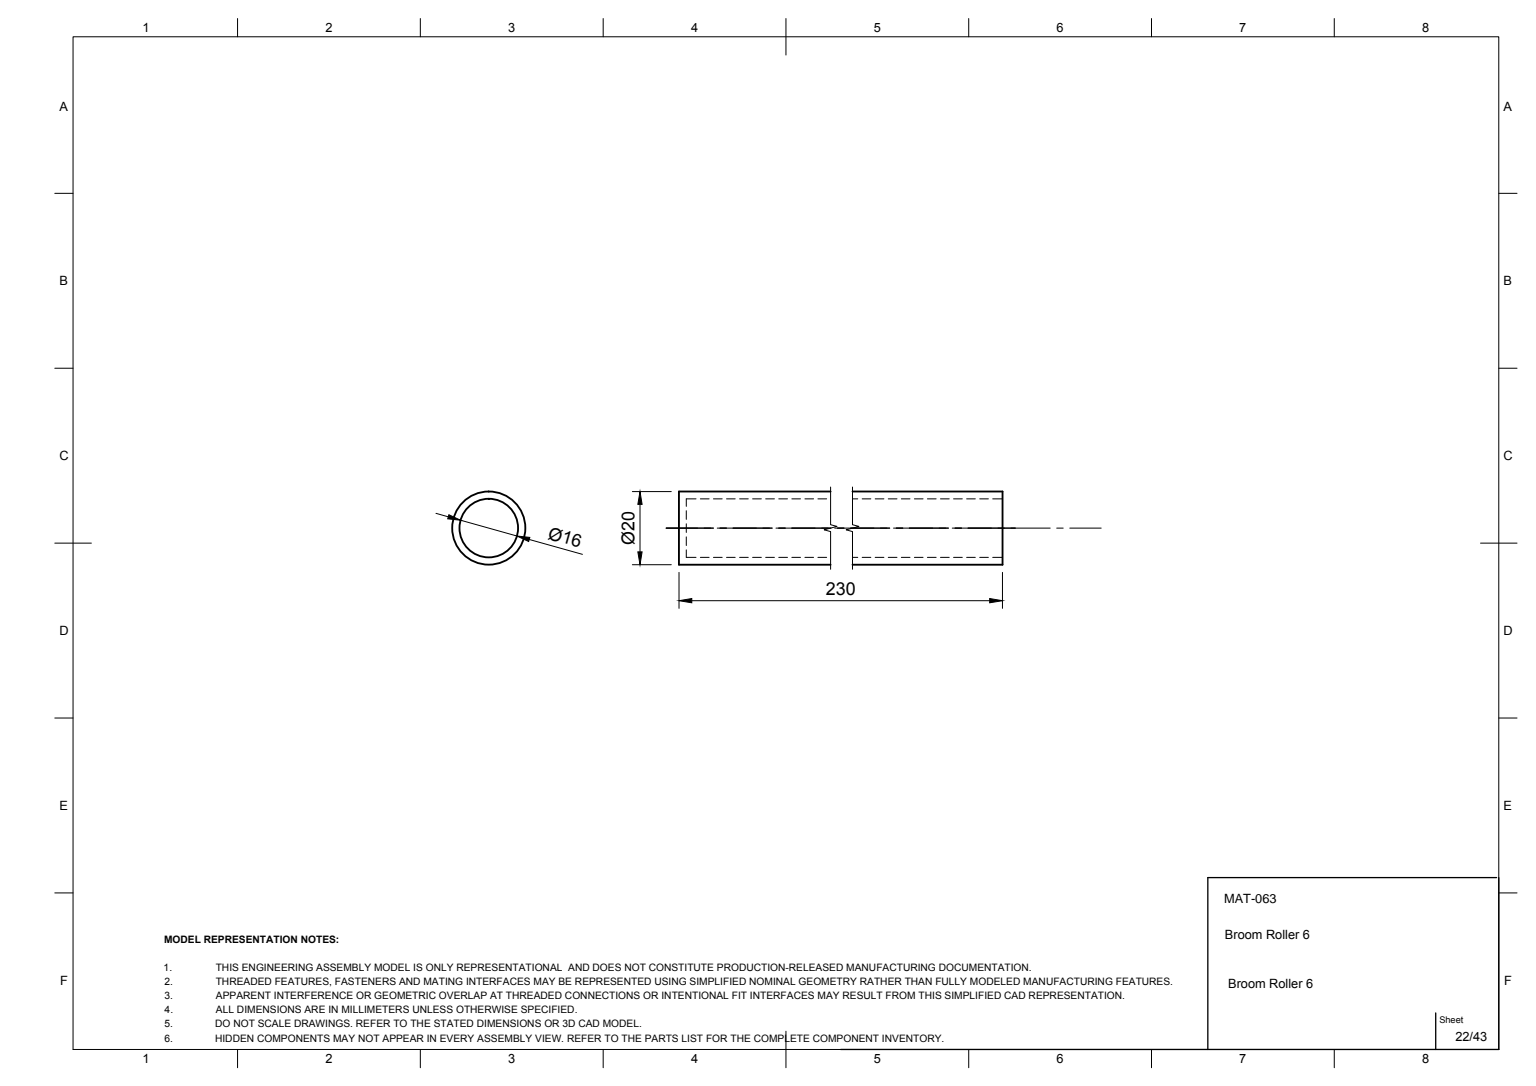
ISO-10303-21;
HEADER;
/* Generated by software containing ST-Developer
 * from STEP Tools, Inc. (www.steptools.com) 
 */

FILE_DESCRIPTION(
/* description */ (''),
/* implementation_level */ '2;1');

FILE_NAME(
/* name */ 'Broom Roller 6.step',
/* time_stamp */ '2026-10-24T09:43:01-07:00',
/* author */ (''),
/* organization */ (''),
/* preprocessor_version */ 'ST-DEVELOPER v20.2',
/* originating_system */ 'Autodesk Translation Framework v15.15.0.0',
/* authorisation */ '');

FILE_SCHEMA (('AUTOMOTIVE_DESIGN { 1 0 10303 214 3 1 1 }'));
ENDSEC;

DATA;
#10=MECHANICAL_DESIGN_GEOMETRIC_PRESENTATION_REPRESENTATION('',(#287),#11112);
#221=SHAPE_REPRESENTATION_RELATIONSHIP('SRR','None',#11245,#254);
#254=ADVANCED_BREP_SHAPE_REPRESENTATION('',(#320),#11090);
#287=STYLED_ITEM('',(#11426),#320);
#320=MANIFOLD_SOLID_BREP('Broom Roller 6',#6024);
#414=FACE_BOUND('',#1328,.T.);
#585=PLANE('',#6918);
#586=PLANE('',#6919);
#587=PLANE('',#6923);
#886=FACE_OUTER_BOUND('',#1325,.T.);
#887=FACE_OUTER_BOUND('',#1326,.T.);
#888=FACE_OUTER_BOUND('',#1327,.T.);
#889=FACE_OUTER_BOUND('',#1329,.T.);
#890=FACE_OUTER_BOUND('',#1330,.T.);
#1325=EDGE_LOOP('',(#4853,#4854,#4855,#4856));
#1326=EDGE_LOOP('',(#4857));
#1327=EDGE_LOOP('',(#4858));
#1328=EDGE_LOOP('',(#4859));
#1329=EDGE_LOOP('',(#4860,#4861,#4862,#4863));
#1330=EDGE_LOOP('',(#4864));
#1730=LINE('',#10291,#2089);
#1731=LINE('',#10300,#2090);
#2089=VECTOR('',#8452,0.00799999974106502);
#2090=VECTOR('',#8465,0.00999999987547767);
#2554=CIRCLE('',#6916,0.00799999974106502);
#2555=CIRCLE('',#6917,0.00799999974106502);
#2556=CIRCLE('',#6920,0.00999999987547767);
#2557=CIRCLE('',#6922,0.00999999987547767);
#2964=VERTEX_POINT('',#10288);
#2965=VERTEX_POINT('',#10290);
#2966=VERTEX_POINT('',#10295);
#2967=VERTEX_POINT('',#10298);
#3630=EDGE_CURVE('',#2964,#2964,#2554,.T.);
#3631=EDGE_CURVE('',#2964,#2965,#1730,.T.);
#3632=EDGE_CURVE('',#2965,#2965,#2555,.F.);
#3633=EDGE_CURVE('',#2966,#2966,#2556,.T.);
#3634=EDGE_CURVE('',#2967,#2967,#2557,.F.);
#3635=EDGE_CURVE('',#2967,#2966,#1731,.T.);
#4853=ORIENTED_EDGE('',*,*,#3630,.F.);
#4854=ORIENTED_EDGE('',*,*,#3631,.T.);
#4855=ORIENTED_EDGE('',*,*,#3632,.F.);
#4856=ORIENTED_EDGE('',*,*,#3631,.F.);
#4857=ORIENTED_EDGE('',*,*,#3632,.T.);
#4858=ORIENTED_EDGE('',*,*,#3633,.F.);
#4859=ORIENTED_EDGE('',*,*,#3630,.T.);
#4860=ORIENTED_EDGE('',*,*,#3634,.T.);
#4861=ORIENTED_EDGE('',*,*,#3635,.T.);
#4862=ORIENTED_EDGE('',*,*,#3633,.T.);
#4863=ORIENTED_EDGE('',*,*,#3635,.F.);
#4864=ORIENTED_EDGE('',*,*,#3634,.F.);
#5575=CYLINDRICAL_SURFACE('',#6915,0.00799999974106502);
#5576=CYLINDRICAL_SURFACE('',#6921,0.00999999987547767);
#5859=ADVANCED_FACE('',(#886),#5575,.F.);
#5860=ADVANCED_FACE('',(#887),#585,.F.);
#5861=ADVANCED_FACE('',(#888,#414),#586,.F.);
#5862=ADVANCED_FACE('',(#889),#5576,.T.);
#5863=ADVANCED_FACE('',(#890),#587,.T.);
#6024=CLOSED_SHELL('',(#5859,#5860,#5861,#5862,#5863));
#6914=AXIS2_PLACEMENT_3D('',#10286,#8446,#8447);
#6915=AXIS2_PLACEMENT_3D('',#10287,#8448,#8449);
#6916=AXIS2_PLACEMENT_3D('',#10289,#8450,#8451);
#6917=AXIS2_PLACEMENT_3D('',#10292,#8453,#8454);
#6918=AXIS2_PLACEMENT_3D('',#10293,#8455,#8456);
#6919=AXIS2_PLACEMENT_3D('',#10294,#8457,#8458);
#6920=AXIS2_PLACEMENT_3D('',#10296,#8459,#8460);
#6921=AXIS2_PLACEMENT_3D('',#10297,#8461,#8462);
#6922=AXIS2_PLACEMENT_3D('',#10299,#8463,#8464);
#6923=AXIS2_PLACEMENT_3D('',#10301,#8466,#8467);
#8446=DIRECTION('axis',(0.,0.,1.));
#8447=DIRECTION('refdir',(1.,0.,0.));
#8448=DIRECTION('center_axis',(0.,-0.604097518460404,-0.796910401607346));
#8449=DIRECTION('ref_axis',(0.,0.796910401607346,-0.604097518460404));
#8450=DIRECTION('center_axis',(0.,-0.604097518460404,-0.796910401607346));
#8451=DIRECTION('ref_axis',(0.,0.796910401607346,-0.604097518460404));
#8452=DIRECTION('',(0.,-0.604097518460404,-0.796910401607346));
#8453=DIRECTION('center_axis',(0.,-0.604097518460404,-0.796910401607346));
#8454=DIRECTION('ref_axis',(0.,0.796910401607346,-0.604097518460404));
#8455=DIRECTION('center_axis',(-1.20725909381357E-16,-0.6040974946122,-0.796910419685465));
#8456=DIRECTION('ref_axis',(7.15152886696226E-32,0.796910419685465,-0.6040974946122));
#8457=DIRECTION('center_axis',(6.24224782272207E-17,-0.604097506757326,
-0.796910410478859));
#8458=DIRECTION('ref_axis',(-1.64388262168888E-33,0.796910410478859,-0.604097506757326));
#8459=DIRECTION('center_axis',(0.,-0.604097518460408,-0.796910401607343));
#8460=DIRECTION('ref_axis',(0.,0.796910401607343,-0.604097518460408));
#8461=DIRECTION('center_axis',(0.,-0.604097518460408,-0.796910401607343));
#8462=DIRECTION('ref_axis',(0.,0.796910401607343,-0.604097518460408));
#8463=DIRECTION('center_axis',(0.,-0.604097518460408,-0.796910401607343));
#8464=DIRECTION('ref_axis',(0.,0.796910401607343,-0.604097518460408));
#8465=DIRECTION('',(0.,0.604097518460408,0.796910401607343));
#8466=DIRECTION('center_axis',(-2.35801524345747E-16,-0.604097538134134,
-0.796910386693685));
#8467=DIRECTION('ref_axis',(2.53292576583338E-33,0.796910386693685,-0.604097538134134));
#10286=CARTESIAN_POINT('',(0.,0.,0.));
#10287=CARTESIAN_POINT('Origin',(0.,0.488942429,1.283289392));
#10288=CARTESIAN_POINT('',(-9.79717407607493E-19,0.482567145986908,1.28812217198258));
#10289=CARTESIAN_POINT('Origin',(0.,0.488942428993417,1.28328939199132));
#10290=CARTESIAN_POINT('',(-9.79717407607493E-19,0.344832912126902,1.10642660087645));
#10291=CARTESIAN_POINT('',(-9.79717407607493E-19,0.482567145993489,1.28812217199126));
#10292=CARTESIAN_POINT('Origin',(0.,0.351208195133414,1.10159382088519));
#10293=CARTESIAN_POINT('Origin',(-1.99493199737333E-19,0.351208195,1.1015938205));
#10294=CARTESIAN_POINT('Origin',(-1.56125112837913E-19,0.488942429,1.2832893925));
#10295=CARTESIAN_POINT('',(-1.22464678389777E-18,0.480973325166166,1.28933036721888));
#10296=CARTESIAN_POINT('Origin',(0.,0.488942429083005,1.2832893921095));
#10297=CARTESIAN_POINT('Origin',(0.,0.488942429,1.283289392));
#10298=CARTESIAN_POINT('',(-1.22464678389777E-18,0.342030896187977,1.10604097520234));
#10299=CARTESIAN_POINT('Origin',(0.,0.350000000104818,1.10000000009296));
#10300=CARTESIAN_POINT('',(-1.22464678389777E-18,0.48097332508316,1.28933036710938));
#10301=CARTESIAN_POINT('Origin',(-1.56125112837913E-19,0.35,1.1));
#11051=UNCERTAINTY_MEASURE_WITH_UNIT(LENGTH_MEASURE(1.E-5),#11113,
'DISTANCE_ACCURACY_VALUE',
'Maximum model space distance between geometric entities at asserted c
onnectivities');
#11073=UNCERTAINTY_MEASURE_WITH_UNIT(LENGTH_MEASURE(1.E-5),#11113,
'DISTANCE_ACCURACY_VALUE',
'Maximum model space distance between geometric entities at asserted c
onnectivities');
#11090=(
GEOMETRIC_REPRESENTATION_CONTEXT(3)
GLOBAL_UNCERTAINTY_ASSIGNED_CONTEXT((#11051))
GLOBAL_UNIT_ASSIGNED_CONTEXT((#11113,#11114,#11115))
REPRESENTATION_CONTEXT('','3D')
);
#11112=(
GEOMETRIC_REPRESENTATION_CONTEXT(3)
GLOBAL_UNCERTAINTY_ASSIGNED_CONTEXT((#11073))
GLOBAL_UNIT_ASSIGNED_CONTEXT((#11113,#11114,#11115))
REPRESENTATION_CONTEXT('','3D')
);
#11113=(
LENGTH_UNIT()
NAMED_UNIT(*)
SI_UNIT($,.METRE.)
);
#11114=(
NAMED_UNIT(*)
PLANE_ANGLE_UNIT()
SI_UNIT($,.RADIAN.)
);
#11115=(
NAMED_UNIT(*)
SI_UNIT($,.STERADIAN.)
SOLID_ANGLE_UNIT()
);
#11132=SHAPE_DEFINITION_REPRESENTATION(#11170,#11245);
#11170=PRODUCT_DEFINITION_SHAPE('',$,#11284);
#11245=SHAPE_REPRESENTATION('',(#6914),#11090);
#11267=PRODUCT_DEFINITION_CONTEXT('part definition',#11383,'design');
#11284=PRODUCT_DEFINITION('Broom Roller 6','Broom Roller 6',#11322,#11267);
#11322=PRODUCT_DEFINITION_FORMATION('',$,#11401);
#11383=APPLICATION_CONTEXT(
'Core Data for Automotive Mechanical Design Process');
#11384=PRODUCT_CONTEXT('part definition',#11383,'mechanical');
#11401=PRODUCT('Broom Roller 6','Broom Roller 6',
'broom_and_roller__ DE     6985',(#11384));
#11426=PRESENTATION_STYLE_ASSIGNMENT((#11430));
#11430=SURFACE_STYLE_USAGE(.BOTH.,#11434);
#11434=SURFACE_SIDE_STYLE('',(#11438));
#11438=SURFACE_STYLE_FILL_AREA(#11442);
#11442=FILL_AREA_STYLE('Opaque(202,209,238)',(#11446));
#11446=FILL_AREA_STYLE_COLOUR('Opaque(202,209,238)',#11450);
#11450=COLOUR_RGB('Opaque(202,209,238)',0.792156862745098,0.819607843137255,
0.933333333333333);
ENDSEC;
END-ISO-10303-21;
